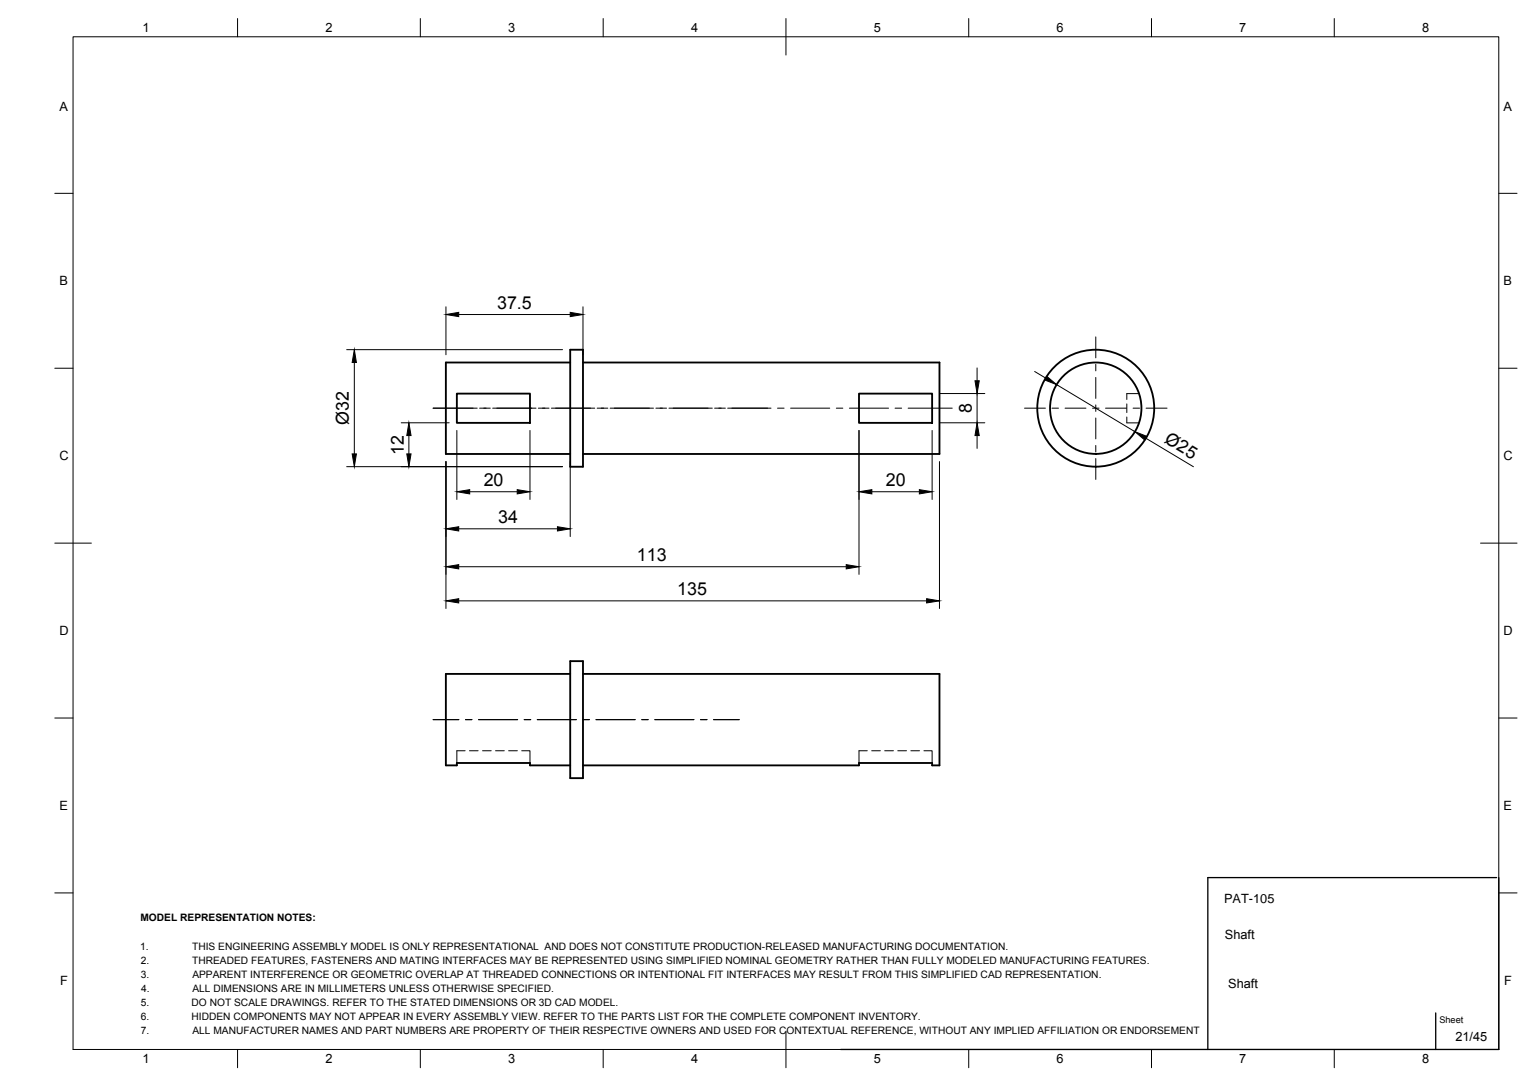
ISO-10303-21;
HEADER;
/* Generated by software containing ST-Developer
 * from STEP Tools, Inc. (www.steptools.com) 
 */

FILE_DESCRIPTION(
/* description */ ('Torque wrench calibration arm'),
/* implementation_level */ '2;1');

FILE_NAME(
/* name */ 'Shaft.step',
/* time_stamp */ '2026-10-28T03:24:52-07:00',
/* author */ (''),
/* organization */ (''),
/* preprocessor_version */ 'ST-DEVELOPER v20.2',
/* originating_system */ 'Autodesk Translation Framework v15.17.0.0',
/* authorisation */ '');

FILE_SCHEMA (('AUTOMOTIVE_DESIGN { 1 0 10303 214 3 1 1 }'));
ENDSEC;

DATA;
#10=MECHANICAL_DESIGN_GEOMETRIC_PRESENTATION_REPRESENTATION('',(#449),#12783);
#366=SHAPE_REPRESENTATION_RELATIONSHIP('SRR','None',#12949,#403);
#403=ADVANCED_BREP_SHAPE_REPRESENTATION('',(#501),#12758);
#449=STYLED_ITEM('',(#13212),#501);
#501=MANIFOLD_SOLID_BREP('Body1',#6520);
#594=FACE_BOUND('',#1532,.T.);
#595=FACE_BOUND('',#1534,.T.);
#596=FACE_BOUND('',#1537,.T.);
#597=FACE_BOUND('',#1539,.T.);
#750=PLANE('',#7376);
#751=PLANE('',#7377);
#752=PLANE('',#7379);
#753=PLANE('',#7380);
#754=PLANE('',#7381);
#755=PLANE('',#7383);
#756=PLANE('',#7384);
#757=PLANE('',#7386);
#758=PLANE('',#7387);
#759=PLANE('',#7388);
#760=PLANE('',#7390);
#761=PLANE('',#7393);
#762=PLANE('',#7401);
#763=PLANE('',#7402);
#1063=FACE_OUTER_BOUND('',#1521,.T.);
#1064=FACE_OUTER_BOUND('',#1522,.T.);
#1065=FACE_OUTER_BOUND('',#1523,.T.);
#1066=FACE_OUTER_BOUND('',#1524,.T.);
#1067=FACE_OUTER_BOUND('',#1525,.T.);
#1068=FACE_OUTER_BOUND('',#1526,.T.);
#1069=FACE_OUTER_BOUND('',#1527,.T.);
#1070=FACE_OUTER_BOUND('',#1528,.T.);
#1071=FACE_OUTER_BOUND('',#1529,.T.);
#1072=FACE_OUTER_BOUND('',#1530,.T.);
#1073=FACE_OUTER_BOUND('',#1531,.T.);
#1074=FACE_OUTER_BOUND('',#1533,.T.);
#1075=FACE_OUTER_BOUND('',#1535,.T.);
#1076=FACE_OUTER_BOUND('',#1536,.T.);
#1077=FACE_OUTER_BOUND('',#1538,.T.);
#1078=FACE_OUTER_BOUND('',#1540,.T.);
#1079=FACE_OUTER_BOUND('',#1541,.T.);
#1521=EDGE_LOOP('',(#5149,#5150,#5151,#5152));
#1522=EDGE_LOOP('',(#5153,#5154,#5155,#5156));
#1523=EDGE_LOOP('',(#5157,#5158,#5159,#5160));
#1524=EDGE_LOOP('',(#5161,#5162,#5163,#5164));
#1525=EDGE_LOOP('',(#5165,#5166,#5167,#5168));
#1526=EDGE_LOOP('',(#5169,#5170,#5171,#5172));
#1527=EDGE_LOOP('',(#5173,#5174,#5175,#5176));
#1528=EDGE_LOOP('',(#5177,#5178,#5179,#5180));
#1529=EDGE_LOOP('',(#5181,#5182,#5183,#5184));
#1530=EDGE_LOOP('',(#5185,#5186,#5187,#5188));
#1531=EDGE_LOOP('',(#5189));
#1532=EDGE_LOOP('',(#5190));
#1533=EDGE_LOOP('',(#5191));
#1534=EDGE_LOOP('',(#5192));
#1535=EDGE_LOOP('',(#5193,#5194,#5195,#5196));
#1536=EDGE_LOOP('',(#5197,#5198,#5199,#5200));
#1537=EDGE_LOOP('',(#5201,#5202,#5203,#5204));
#1538=EDGE_LOOP('',(#5205,#5206,#5207,#5208));
#1539=EDGE_LOOP('',(#5209,#5210,#5211,#5212));
#1540=EDGE_LOOP('',(#5213));
#1541=EDGE_LOOP('',(#5214));
#1984=LINE('',#11212,#2399);
#1985=LINE('',#11214,#2400);
#1986=LINE('',#11216,#2401);
#1987=LINE('',#11217,#2402);
#1988=LINE('',#11222,#2403);
#1989=LINE('',#11223,#2404);
#1990=LINE('',#11226,#2405);
#1991=LINE('',#11228,#2406);
#1992=LINE('',#11229,#2407);
#1993=LINE('',#11231,#2408);
#1994=LINE('',#11237,#2409);
#1995=LINE('',#11239,#2410);
#1996=LINE('',#11241,#2411);
#1997=LINE('',#11242,#2412);
#1998=LINE('',#11247,#2413);
#1999=LINE('',#11248,#2414);
#2000=LINE('',#11251,#2415);
#2001=LINE('',#11253,#2416);
#2002=LINE('',#11254,#2417);
#2003=LINE('',#11256,#2418);
#2004=LINE('',#11270,#2419);
#2005=LINE('',#11273,#2420);
#2006=LINE('',#11278,#2421);
#2399=VECTOR('',#8842,1.);
#2400=VECTOR('',#8843,1.);
#2401=VECTOR('',#8844,1.);
#2402=VECTOR('',#8845,1.);
#2403=VECTOR('',#8850,1.);
#2404=VECTOR('',#8851,1.);
#2405=VECTOR('',#8854,1.);
#2406=VECTOR('',#8855,1.);
#2407=VECTOR('',#8856,1.);
#2408=VECTOR('',#8859,1.);
#2409=VECTOR('',#8866,1.);
#2410=VECTOR('',#8867,1.);
#2411=VECTOR('',#8868,1.);
#2412=VECTOR('',#8869,1.);
#2413=VECTOR('',#8874,1.);
#2414=VECTOR('',#8875,1.);
#2415=VECTOR('',#8878,1.);
#2416=VECTOR('',#8879,1.);
#2417=VECTOR('',#8880,1.);
#2418=VECTOR('',#8883,1.);
#2419=VECTOR('',#8902,1.6);
#2420=VECTOR('',#8905,1.25);
#2421=VECTOR('',#8912,1.25);
#2799=CIRCLE('',#7378,1.25);
#2800=CIRCLE('',#7382,1.25);
#2801=CIRCLE('',#7385,1.25);
#2802=CIRCLE('',#7389,1.25);
#2803=CIRCLE('',#7391,1.6);
#2804=CIRCLE('',#7392,1.25);
#2805=CIRCLE('',#7394,1.6);
#2806=CIRCLE('',#7395,1.25);
#2807=CIRCLE('',#7398,1.25);
#2808=CIRCLE('',#7400,1.25);
#3245=VERTEX_POINT('',#11210);
#3246=VERTEX_POINT('',#11211);
#3247=VERTEX_POINT('',#11213);
#3248=VERTEX_POINT('',#11215);
#3249=VERTEX_POINT('',#11219);
#3250=VERTEX_POINT('',#11221);
#3251=VERTEX_POINT('',#11225);
#3252=VERTEX_POINT('',#11227);
#3253=VERTEX_POINT('',#11235);
#3254=VERTEX_POINT('',#11236);
#3255=VERTEX_POINT('',#11238);
#3256=VERTEX_POINT('',#11240);
#3257=VERTEX_POINT('',#11244);
#3258=VERTEX_POINT('',#11246);
#3259=VERTEX_POINT('',#11250);
#3260=VERTEX_POINT('',#11252);
#3261=VERTEX_POINT('',#11260);
#3262=VERTEX_POINT('',#11262);
#3263=VERTEX_POINT('',#11265);
#3264=VERTEX_POINT('',#11267);
#3265=VERTEX_POINT('',#11272);
#3266=VERTEX_POINT('',#11276);
#3932=EDGE_CURVE('',#3245,#3246,#1984,.T.);
#3933=EDGE_CURVE('',#3245,#3247,#1985,.T.);
#3934=EDGE_CURVE('',#3248,#3247,#1986,.T.);
#3935=EDGE_CURVE('',#3248,#3246,#1987,.T.);
#3936=EDGE_CURVE('',#3246,#3249,#2799,.T.);
#3937=EDGE_CURVE('',#3250,#3248,#1988,.T.);
#3938=EDGE_CURVE('',#3249,#3250,#1989,.T.);
#3939=EDGE_CURVE('',#3249,#3251,#1990,.T.);
#3940=EDGE_CURVE('',#3250,#3252,#1991,.T.);
#3941=EDGE_CURVE('',#3252,#3251,#1992,.T.);
#3942=EDGE_CURVE('',#3247,#3252,#1993,.T.);
#3943=EDGE_CURVE('',#3251,#3245,#2800,.T.);
#3944=EDGE_CURVE('',#3253,#3254,#1994,.T.);
#3945=EDGE_CURVE('',#3253,#3255,#1995,.T.);
#3946=EDGE_CURVE('',#3256,#3255,#1996,.T.);
#3947=EDGE_CURVE('',#3256,#3254,#1997,.T.);
#3948=EDGE_CURVE('',#3254,#3257,#2801,.T.);
#3949=EDGE_CURVE('',#3258,#3256,#1998,.T.);
#3950=EDGE_CURVE('',#3257,#3258,#1999,.T.);
#3951=EDGE_CURVE('',#3257,#3259,#2000,.T.);
#3952=EDGE_CURVE('',#3258,#3260,#2001,.T.);
#3953=EDGE_CURVE('',#3260,#3259,#2002,.T.);
#3954=EDGE_CURVE('',#3255,#3260,#2003,.T.);
#3955=EDGE_CURVE('',#3259,#3253,#2802,.T.);
#3956=EDGE_CURVE('',#3261,#3261,#2803,.T.);
#3957=EDGE_CURVE('',#3262,#3262,#2804,.T.);
#3958=EDGE_CURVE('',#3263,#3263,#2805,.T.);
#3959=EDGE_CURVE('',#3264,#3264,#2806,.T.);
#3960=EDGE_CURVE('',#3261,#3263,#2004,.T.);
#3961=EDGE_CURVE('',#3264,#3265,#2005,.T.);
#3962=EDGE_CURVE('',#3265,#3265,#2807,.T.);
#3963=EDGE_CURVE('',#3266,#3266,#2808,.T.);
#3964=EDGE_CURVE('',#3266,#3262,#2006,.T.);
#5149=ORIENTED_EDGE('',*,*,#3932,.F.);
#5150=ORIENTED_EDGE('',*,*,#3933,.T.);
#5151=ORIENTED_EDGE('',*,*,#3934,.F.);
#5152=ORIENTED_EDGE('',*,*,#3935,.T.);
#5153=ORIENTED_EDGE('',*,*,#3936,.F.);
#5154=ORIENTED_EDGE('',*,*,#3935,.F.);
#5155=ORIENTED_EDGE('',*,*,#3937,.F.);
#5156=ORIENTED_EDGE('',*,*,#3938,.F.);
#5157=ORIENTED_EDGE('',*,*,#3939,.F.);
#5158=ORIENTED_EDGE('',*,*,#3938,.T.);
#5159=ORIENTED_EDGE('',*,*,#3940,.T.);
#5160=ORIENTED_EDGE('',*,*,#3941,.T.);
#5161=ORIENTED_EDGE('',*,*,#3937,.T.);
#5162=ORIENTED_EDGE('',*,*,#3934,.T.);
#5163=ORIENTED_EDGE('',*,*,#3942,.T.);
#5164=ORIENTED_EDGE('',*,*,#3940,.F.);
#5165=ORIENTED_EDGE('',*,*,#3943,.F.);
#5166=ORIENTED_EDGE('',*,*,#3941,.F.);
#5167=ORIENTED_EDGE('',*,*,#3942,.F.);
#5168=ORIENTED_EDGE('',*,*,#3933,.F.);
#5169=ORIENTED_EDGE('',*,*,#3944,.F.);
#5170=ORIENTED_EDGE('',*,*,#3945,.T.);
#5171=ORIENTED_EDGE('',*,*,#3946,.F.);
#5172=ORIENTED_EDGE('',*,*,#3947,.T.);
#5173=ORIENTED_EDGE('',*,*,#3948,.F.);
#5174=ORIENTED_EDGE('',*,*,#3947,.F.);
#5175=ORIENTED_EDGE('',*,*,#3949,.F.);
#5176=ORIENTED_EDGE('',*,*,#3950,.F.);
#5177=ORIENTED_EDGE('',*,*,#3951,.F.);
#5178=ORIENTED_EDGE('',*,*,#3950,.T.);
#5179=ORIENTED_EDGE('',*,*,#3952,.T.);
#5180=ORIENTED_EDGE('',*,*,#3953,.T.);
#5181=ORIENTED_EDGE('',*,*,#3949,.T.);
#5182=ORIENTED_EDGE('',*,*,#3946,.T.);
#5183=ORIENTED_EDGE('',*,*,#3954,.T.);
#5184=ORIENTED_EDGE('',*,*,#3952,.F.);
#5185=ORIENTED_EDGE('',*,*,#3955,.F.);
#5186=ORIENTED_EDGE('',*,*,#3953,.F.);
#5187=ORIENTED_EDGE('',*,*,#3954,.F.);
#5188=ORIENTED_EDGE('',*,*,#3945,.F.);
#5189=ORIENTED_EDGE('',*,*,#3956,.T.);
#5190=ORIENTED_EDGE('',*,*,#3957,.F.);
#5191=ORIENTED_EDGE('',*,*,#3958,.F.);
#5192=ORIENTED_EDGE('',*,*,#3959,.F.);
#5193=ORIENTED_EDGE('',*,*,#3956,.F.);
#5194=ORIENTED_EDGE('',*,*,#3960,.T.);
#5195=ORIENTED_EDGE('',*,*,#3958,.T.);
#5196=ORIENTED_EDGE('',*,*,#3960,.F.);
#5197=ORIENTED_EDGE('',*,*,#3959,.T.);
#5198=ORIENTED_EDGE('',*,*,#3961,.T.);
#5199=ORIENTED_EDGE('',*,*,#3962,.T.);
#5200=ORIENTED_EDGE('',*,*,#3961,.F.);
#5201=ORIENTED_EDGE('',*,*,#3951,.T.);
#5202=ORIENTED_EDGE('',*,*,#3955,.T.);
#5203=ORIENTED_EDGE('',*,*,#3944,.T.);
#5204=ORIENTED_EDGE('',*,*,#3948,.T.);
#5205=ORIENTED_EDGE('',*,*,#3963,.F.);
#5206=ORIENTED_EDGE('',*,*,#3964,.T.);
#5207=ORIENTED_EDGE('',*,*,#3957,.T.);
#5208=ORIENTED_EDGE('',*,*,#3964,.F.);
#5209=ORIENTED_EDGE('',*,*,#3939,.T.);
#5210=ORIENTED_EDGE('',*,*,#3943,.T.);
#5211=ORIENTED_EDGE('',*,*,#3932,.T.);
#5212=ORIENTED_EDGE('',*,*,#3936,.T.);
#5213=ORIENTED_EDGE('',*,*,#3963,.T.);
#5214=ORIENTED_EDGE('',*,*,#3962,.F.);
#6045=CYLINDRICAL_SURFACE('',#7396,1.6);
#6046=CYLINDRICAL_SURFACE('',#7397,1.25);
#6047=CYLINDRICAL_SURFACE('',#7399,1.25);
#6288=ADVANCED_FACE('',(#1063),#750,.F.);
#6289=ADVANCED_FACE('',(#1064),#751,.T.);
#6290=ADVANCED_FACE('',(#1065),#752,.F.);
#6291=ADVANCED_FACE('',(#1066),#753,.F.);
#6292=ADVANCED_FACE('',(#1067),#754,.F.);
#6293=ADVANCED_FACE('',(#1068),#755,.F.);
#6294=ADVANCED_FACE('',(#1069),#756,.T.);
#6295=ADVANCED_FACE('',(#1070),#757,.F.);
#6296=ADVANCED_FACE('',(#1071),#758,.F.);
#6297=ADVANCED_FACE('',(#1072),#759,.F.);
#6298=ADVANCED_FACE('',(#1073,#594),#760,.T.);
#6299=ADVANCED_FACE('',(#1074,#595),#761,.F.);
#6300=ADVANCED_FACE('',(#1075),#6045,.T.);
#6301=ADVANCED_FACE('',(#1076,#596),#6046,.T.);
#6302=ADVANCED_FACE('',(#1077,#597),#6047,.T.);
#6303=ADVANCED_FACE('',(#1078),#762,.T.);
#6304=ADVANCED_FACE('',(#1079),#763,.F.);
#6520=CLOSED_SHELL('',(#6288,#6289,#6290,#6291,#6292,#6293,#6294,#6295,
#6296,#6297,#6298,#6299,#6300,#6301,#6302,#6303,#6304));
#7375=AXIS2_PLACEMENT_3D('',#11208,#8838,#8839);
#7376=AXIS2_PLACEMENT_3D('',#11209,#8840,#8841);
#7377=AXIS2_PLACEMENT_3D('',#11218,#8846,#8847);
#7378=AXIS2_PLACEMENT_3D('',#11220,#8848,#8849);
#7379=AXIS2_PLACEMENT_3D('',#11224,#8852,#8853);
#7380=AXIS2_PLACEMENT_3D('',#11230,#8857,#8858);
#7381=AXIS2_PLACEMENT_3D('',#11232,#8860,#8861);
#7382=AXIS2_PLACEMENT_3D('',#11233,#8862,#8863);
#7383=AXIS2_PLACEMENT_3D('',#11234,#8864,#8865);
#7384=AXIS2_PLACEMENT_3D('',#11243,#8870,#8871);
#7385=AXIS2_PLACEMENT_3D('',#11245,#8872,#8873);
#7386=AXIS2_PLACEMENT_3D('',#11249,#8876,#8877);
#7387=AXIS2_PLACEMENT_3D('',#11255,#8881,#8882);
#7388=AXIS2_PLACEMENT_3D('',#11257,#8884,#8885);
#7389=AXIS2_PLACEMENT_3D('',#11258,#8886,#8887);
#7390=AXIS2_PLACEMENT_3D('',#11259,#8888,#8889);
#7391=AXIS2_PLACEMENT_3D('',#11261,#8890,#8891);
#7392=AXIS2_PLACEMENT_3D('',#11263,#8892,#8893);
#7393=AXIS2_PLACEMENT_3D('',#11264,#8894,#8895);
#7394=AXIS2_PLACEMENT_3D('',#11266,#8896,#8897);
#7395=AXIS2_PLACEMENT_3D('',#11268,#8898,#8899);
#7396=AXIS2_PLACEMENT_3D('',#11269,#8900,#8901);
#7397=AXIS2_PLACEMENT_3D('',#11271,#8903,#8904);
#7398=AXIS2_PLACEMENT_3D('',#11274,#8906,#8907);
#7399=AXIS2_PLACEMENT_3D('',#11275,#8908,#8909);
#7400=AXIS2_PLACEMENT_3D('',#11277,#8910,#8911);
#7401=AXIS2_PLACEMENT_3D('',#11279,#8913,#8914);
#7402=AXIS2_PLACEMENT_3D('',#11280,#8915,#8916);
#8838=DIRECTION('axis',(0.,0.,1.));
#8839=DIRECTION('refdir',(1.,0.,0.));
#8840=DIRECTION('center_axis',(-1.,0.,0.));
#8841=DIRECTION('ref_axis',(0.,0.,1.));
#8842=DIRECTION('',(0.,-1.,0.));
#8843=DIRECTION('',(0.,0.,1.));
#8844=DIRECTION('',(0.,1.,0.));
#8845=DIRECTION('',(0.,0.,-1.));
#8846=DIRECTION('center_axis',(0.,1.,0.));
#8847=DIRECTION('ref_axis',(1.,0.,0.));
#8848=DIRECTION('center_axis',(0.,-1.,0.));
#8849=DIRECTION('ref_axis',(1.,0.,0.));
#8850=DIRECTION('',(-1.,0.,0.));
#8851=DIRECTION('',(0.,0.,1.));
#8852=DIRECTION('center_axis',(1.,0.,0.));
#8853=DIRECTION('ref_axis',(0.,0.,-1.));
#8854=DIRECTION('',(0.,1.,0.));
#8855=DIRECTION('',(0.,1.,0.));
#8856=DIRECTION('',(0.,0.,-1.));
#8857=DIRECTION('center_axis',(0.,0.,1.));
#8858=DIRECTION('ref_axis',(1.,0.,0.));
#8859=DIRECTION('',(1.,0.,0.));
#8860=DIRECTION('center_axis',(0.,1.,0.));
#8861=DIRECTION('ref_axis',(0.,0.,1.));
#8862=DIRECTION('center_axis',(0.,1.,0.));
#8863=DIRECTION('ref_axis',(1.,0.,0.));
#8864=DIRECTION('center_axis',(-1.,0.,0.));
#8865=DIRECTION('ref_axis',(0.,0.,1.));
#8866=DIRECTION('',(0.,-1.,0.));
#8867=DIRECTION('',(0.,0.,1.));
#8868=DIRECTION('',(0.,1.,0.));
#8869=DIRECTION('',(0.,0.,-1.));
#8870=DIRECTION('center_axis',(0.,1.,0.));
#8871=DIRECTION('ref_axis',(1.,0.,0.));
#8872=DIRECTION('center_axis',(0.,-1.,0.));
#8873=DIRECTION('ref_axis',(1.,0.,0.));
#8874=DIRECTION('',(-1.,0.,0.));
#8875=DIRECTION('',(0.,0.,1.));
#8876=DIRECTION('center_axis',(1.,0.,0.));
#8877=DIRECTION('ref_axis',(0.,0.,-1.));
#8878=DIRECTION('',(0.,1.,0.));
#8879=DIRECTION('',(0.,1.,0.));
#8880=DIRECTION('',(0.,0.,-1.));
#8881=DIRECTION('center_axis',(0.,0.,1.));
#8882=DIRECTION('ref_axis',(1.,0.,0.));
#8883=DIRECTION('',(1.,0.,0.));
#8884=DIRECTION('center_axis',(0.,1.,0.));
#8885=DIRECTION('ref_axis',(0.,0.,1.));
#8886=DIRECTION('center_axis',(0.,1.,0.));
#8887=DIRECTION('ref_axis',(1.,0.,0.));
#8888=DIRECTION('center_axis',(0.,1.,0.));
#8889=DIRECTION('ref_axis',(1.,0.,0.));
#8890=DIRECTION('center_axis',(0.,1.,0.));
#8891=DIRECTION('ref_axis',(1.,0.,0.));
#8892=DIRECTION('center_axis',(0.,1.,0.));
#8893=DIRECTION('ref_axis',(1.,0.,0.));
#8894=DIRECTION('center_axis',(0.,1.,0.));
#8895=DIRECTION('ref_axis',(1.,0.,0.));
#8896=DIRECTION('center_axis',(0.,1.,0.));
#8897=DIRECTION('ref_axis',(1.,0.,0.));
#8898=DIRECTION('center_axis',(0.,-1.,0.));
#8899=DIRECTION('ref_axis',(1.,0.,0.));
#8900=DIRECTION('center_axis',(0.,1.,0.));
#8901=DIRECTION('ref_axis',(1.,0.,0.));
#8902=DIRECTION('',(0.,-1.,0.));
#8903=DIRECTION('center_axis',(0.,1.,0.));
#8904=DIRECTION('ref_axis',(1.,0.,0.));
#8905=DIRECTION('',(0.,-1.,0.));
#8906=DIRECTION('center_axis',(0.,1.,0.));
#8907=DIRECTION('ref_axis',(1.,0.,0.));
#8908=DIRECTION('center_axis',(0.,1.,0.));
#8909=DIRECTION('ref_axis',(1.,0.,0.));
#8910=DIRECTION('center_axis',(0.,1.,0.));
#8911=DIRECTION('ref_axis',(1.,0.,0.));
#8912=DIRECTION('',(0.,-1.,0.));
#8913=DIRECTION('center_axis',(0.,1.,0.));
#8914=DIRECTION('ref_axis',(1.,0.,0.));
#8915=DIRECTION('center_axis',(0.,1.,0.));
#8916=DIRECTION('ref_axis',(1.,0.,0.));
#11208=CARTESIAN_POINT('',(0.,0.,0.));
#11209=CARTESIAN_POINT('Origin',(-0.4,7.8,6.6));
#11210=CARTESIAN_POINT('',(-0.4,9.8,6.8157280717673));
#11211=CARTESIAN_POINT('',(-0.4,7.8,6.8157280717673));
#11212=CARTESIAN_POINT('',(-0.4,-3.5,6.8157280717673));
#11213=CARTESIAN_POINT('',(-0.4,9.8,7.15));
#11214=CARTESIAN_POINT('',(-0.4,9.8,7.15));
#11215=CARTESIAN_POINT('',(-0.4,7.8,7.15));
#11216=CARTESIAN_POINT('',(-0.4,7.8,7.15));
#11217=CARTESIAN_POINT('',(-0.4,7.8,7.15));
#11218=CARTESIAN_POINT('Origin',(0.,7.8,6.875));
#11219=CARTESIAN_POINT('',(0.4,7.8,6.8157280717673));
#11220=CARTESIAN_POINT('Origin',(0.,7.8,8.));
#11221=CARTESIAN_POINT('',(0.4,7.8,7.15));
#11222=CARTESIAN_POINT('',(0.4,7.8,7.15));
#11223=CARTESIAN_POINT('',(0.4,7.8,6.6));
#11224=CARTESIAN_POINT('Origin',(0.4,7.8,7.15));
#11225=CARTESIAN_POINT('',(0.4,9.8,6.8157280717673));
#11226=CARTESIAN_POINT('',(0.4,-3.5,6.8157280717673));
#11227=CARTESIAN_POINT('',(0.4,9.8,7.15));
#11228=CARTESIAN_POINT('',(0.4,7.8,7.15));
#11229=CARTESIAN_POINT('',(0.4,9.8,6.6));
#11230=CARTESIAN_POINT('Origin',(-0.4,7.8,7.15));
#11231=CARTESIAN_POINT('',(0.4,9.8,7.15));
#11232=CARTESIAN_POINT('Origin',(0.,9.8,6.875));
#11233=CARTESIAN_POINT('Origin',(0.,9.8,8.));
#11234=CARTESIAN_POINT('Origin',(-0.4,-3.2,6.6));
#11235=CARTESIAN_POINT('',(-0.4,-1.2,6.8157280717673));
#11236=CARTESIAN_POINT('',(-0.4,-3.2,6.8157280717673));
#11237=CARTESIAN_POINT('',(-0.4,-3.5,6.8157280717673));
#11238=CARTESIAN_POINT('',(-0.4,-1.2,7.15));
#11239=CARTESIAN_POINT('',(-0.4,-1.2,7.15));
#11240=CARTESIAN_POINT('',(-0.4,-3.2,7.15));
#11241=CARTESIAN_POINT('',(-0.4,-3.2,7.15));
#11242=CARTESIAN_POINT('',(-0.4,-3.2,7.15));
#11243=CARTESIAN_POINT('Origin',(0.,-3.2,6.875));
#11244=CARTESIAN_POINT('',(0.4,-3.2,6.8157280717673));
#11245=CARTESIAN_POINT('Origin',(0.,-3.2,8.));
#11246=CARTESIAN_POINT('',(0.4,-3.2,7.15));
#11247=CARTESIAN_POINT('',(0.4,-3.2,7.15));
#11248=CARTESIAN_POINT('',(0.4,-3.2,6.6));
#11249=CARTESIAN_POINT('Origin',(0.4,-3.2,7.15));
#11250=CARTESIAN_POINT('',(0.4,-1.2,6.8157280717673));
#11251=CARTESIAN_POINT('',(0.4,-3.5,6.8157280717673));
#11252=CARTESIAN_POINT('',(0.4,-1.2,7.15));
#11253=CARTESIAN_POINT('',(0.4,-3.2,7.15));
#11254=CARTESIAN_POINT('',(0.4,-1.2,6.6));
#11255=CARTESIAN_POINT('Origin',(-0.4,-3.2,7.15));
#11256=CARTESIAN_POINT('',(0.4,-1.2,7.15));
#11257=CARTESIAN_POINT('Origin',(0.,-1.2,6.875));
#11258=CARTESIAN_POINT('Origin',(0.,-1.2,8.));
#11259=CARTESIAN_POINT('Origin',(0.,0.25,8.));
#11260=CARTESIAN_POINT('',(-1.6,0.25,8.));
#11261=CARTESIAN_POINT('Origin',(0.,0.25,8.));
#11262=CARTESIAN_POINT('',(-1.25,0.25,8.));
#11263=CARTESIAN_POINT('Origin',(0.,0.25,8.));
#11264=CARTESIAN_POINT('Origin',(0.,-0.1,8.));
#11265=CARTESIAN_POINT('',(-1.6,-0.1,8.));
#11266=CARTESIAN_POINT('Origin',(0.,-0.1,8.));
#11267=CARTESIAN_POINT('',(-1.25,-0.1,8.));
#11268=CARTESIAN_POINT('Origin',(0.,-0.1,8.));
#11269=CARTESIAN_POINT('Origin',(0.,-0.1,8.));
#11270=CARTESIAN_POINT('',(-1.6,-0.1,8.));
#11271=CARTESIAN_POINT('Origin',(0.,-3.5,8.));
#11272=CARTESIAN_POINT('',(-1.25,-3.5,8.));
#11273=CARTESIAN_POINT('',(-1.25,-3.5,8.));
#11274=CARTESIAN_POINT('Origin',(0.,-3.5,8.));
#11275=CARTESIAN_POINT('Origin',(0.,-3.5,8.));
#11276=CARTESIAN_POINT('',(-1.25,10.,8.));
#11277=CARTESIAN_POINT('Origin',(0.,10.,8.));
#11278=CARTESIAN_POINT('',(-1.25,-3.5,8.));
#11279=CARTESIAN_POINT('Origin',(0.,10.,8.));
#11280=CARTESIAN_POINT('Origin',(0.,-3.5,8.));
#12714=UNCERTAINTY_MEASURE_WITH_UNIT(LENGTH_MEASURE(0.001),#12784,
'DISTANCE_ACCURACY_VALUE',
'Maximum model space distance between geometric entities at asserted c
onnectivities');
#12739=UNCERTAINTY_MEASURE_WITH_UNIT(LENGTH_MEASURE(0.001),#12784,
'DISTANCE_ACCURACY_VALUE',
'Maximum model space distance between geometric entities at asserted c
onnectivities');
#12758=(
GEOMETRIC_REPRESENTATION_CONTEXT(3)
GLOBAL_UNCERTAINTY_ASSIGNED_CONTEXT((#12714))
GLOBAL_UNIT_ASSIGNED_CONTEXT((#12784,#12786,#12787))
REPRESENTATION_CONTEXT('','3D')
);
#12783=(
GEOMETRIC_REPRESENTATION_CONTEXT(3)
GLOBAL_UNCERTAINTY_ASSIGNED_CONTEXT((#12739))
GLOBAL_UNIT_ASSIGNED_CONTEXT((#12784,#12786,#12787))
REPRESENTATION_CONTEXT('','3D')
);
#12784=(
LENGTH_UNIT()
NAMED_UNIT(*)
SI_UNIT(.CENTI.,.METRE.)
);
#12786=(
NAMED_UNIT(*)
PLANE_ANGLE_UNIT()
SI_UNIT($,.RADIAN.)
);
#12787=(
NAMED_UNIT(*)
SI_UNIT($,.STERADIAN.)
SOLID_ANGLE_UNIT()
);
#12806=SHAPE_DEFINITION_REPRESENTATION(#12875,#12949);
#12875=PRODUCT_DEFINITION_SHAPE('',$,#12993);
#12949=SHAPE_REPRESENTATION('',(#7375),#12758);
#12974=PRODUCT_DEFINITION_CONTEXT('part definition',#13105,'design');
#12993=PRODUCT_DEFINITION('Shaft','Shaft',#13036,#12974);
#13036=PRODUCT_DEFINITION_FORMATION('',$,#13125);
#13105=APPLICATION_CONTEXT(
'Core Data for Automotive Mechanical Design Process');
#13106=PRODUCT_CONTEXT('part definition',#13105,'mechanical');
#13125=PRODUCT('Shaft','Shaft','Shaft',(#13106));
#13206=COLOUR_RGB('Grey',0.48,0.52,0.57);
#13207=FILL_AREA_STYLE_COLOUR('',#13206);
#13208=FILL_AREA_STYLE('',(#13207));
#13209=SURFACE_STYLE_FILL_AREA(#13208);
#13210=SURFACE_SIDE_STYLE('',(#13209));
#13211=SURFACE_STYLE_USAGE(.BOTH.,#13210);
#13212=PRESENTATION_STYLE_ASSIGNMENT((#13211));
ENDSEC;
END-ISO-10303-21;
